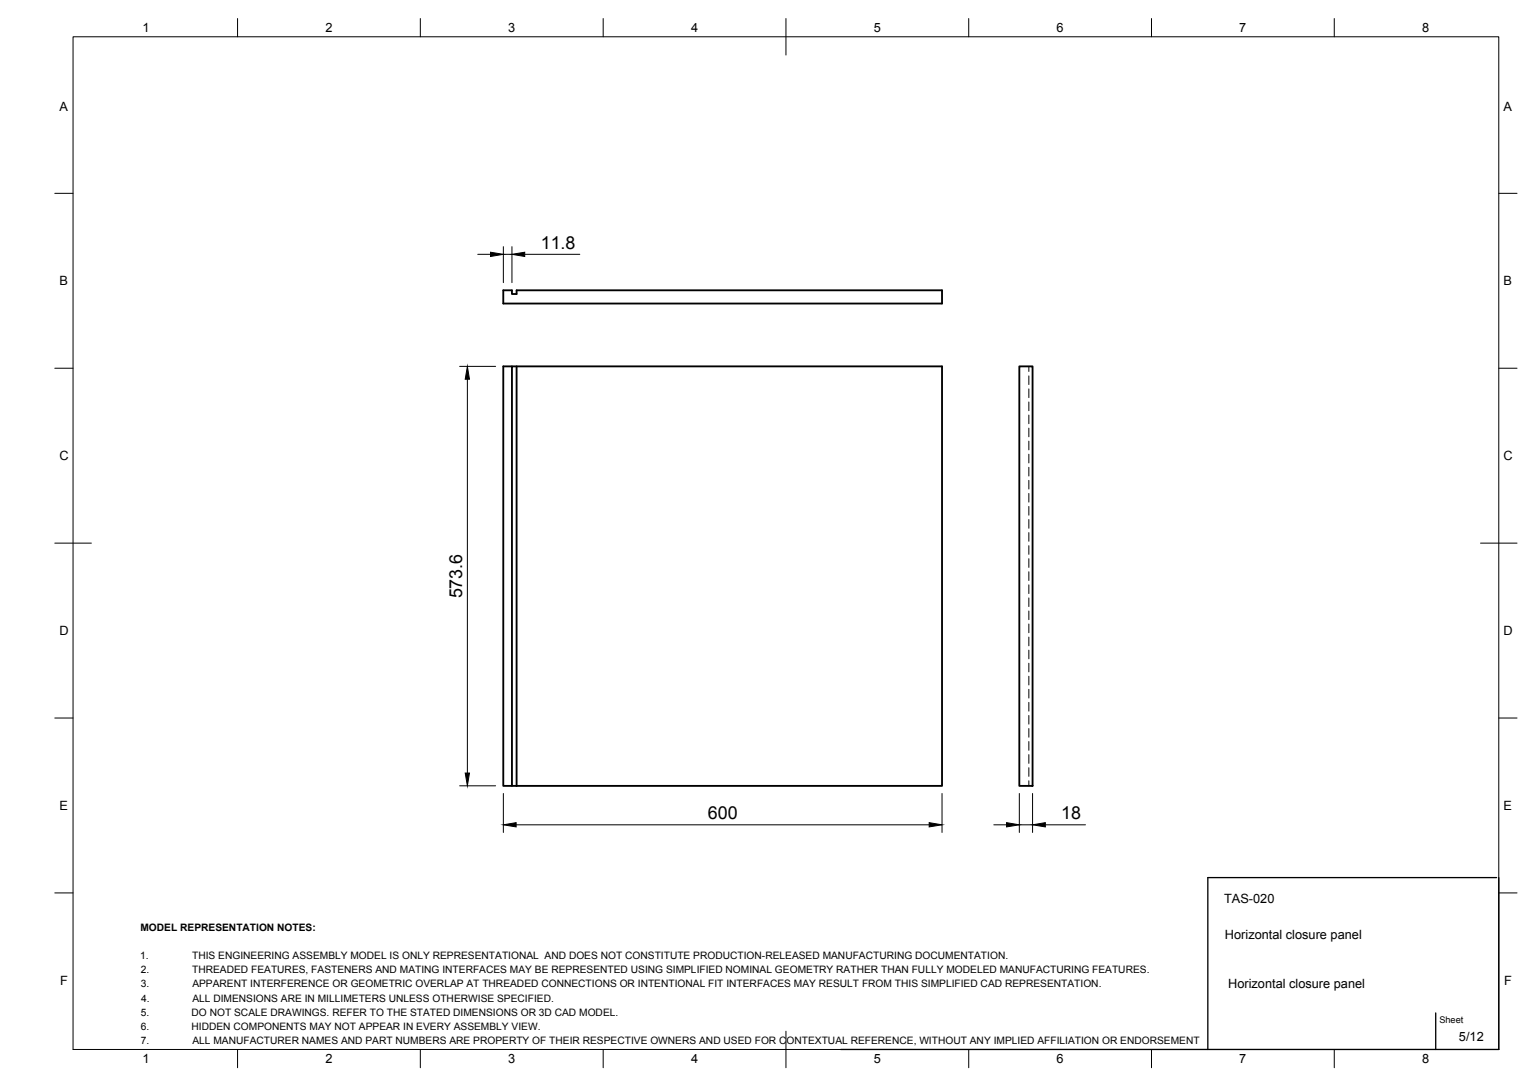
ISO-10303-21;
HEADER;
/* Generated by software containing ST-Developer
 * from STEP Tools, Inc. (www.steptools.com) 
 */

FILE_DESCRIPTION(
/* description */ (''),
/* implementation_level */ '2;1');

FILE_NAME(
/* name */ 'Horizontal closure panel.step',
/* time_stamp */ '2026-11-15T17:46:57-08:00',
/* author */ (''),
/* organization */ (''),
/* preprocessor_version */ 'ST-DEVELOPER v20.2',
/* originating_system */ 'Autodesk Translation Framework v15.17.0.0',
/* authorisation */ '');

FILE_SCHEMA (('AUTOMOTIVE_DESIGN { 1 0 10303 214 3 1 1 }'));
ENDSEC;

DATA;
#10=MECHANICAL_DESIGN_GEOMETRIC_PRESENTATION_REPRESENTATION('',(#377),#12963);
#353=SHAPE_REPRESENTATION_RELATIONSHIP('SRR','None',#13037,#365);
#365=ADVANCED_BREP_SHAPE_REPRESENTATION('',(#389),#12953);
#377=STYLED_ITEM('',(#13106),#389);
#389=MANIFOLD_SOLID_BREP('Body1',#4811);
#495=PLANE('',#5054);
#496=PLANE('',#5055);
#497=PLANE('',#5056);
#498=PLANE('',#5057);
#499=PLANE('',#5058);
#500=PLANE('',#5059);
#501=PLANE('',#5060);
#502=PLANE('',#5061);
#503=PLANE('',#5062);
#504=PLANE('',#5063);
#640=FACE_OUTER_BOUND('',#914,.T.);
#641=FACE_OUTER_BOUND('',#915,.T.);
#642=FACE_OUTER_BOUND('',#916,.T.);
#643=FACE_OUTER_BOUND('',#917,.T.);
#644=FACE_OUTER_BOUND('',#918,.T.);
#645=FACE_OUTER_BOUND('',#919,.T.);
#646=FACE_OUTER_BOUND('',#920,.T.);
#647=FACE_OUTER_BOUND('',#921,.T.);
#648=FACE_OUTER_BOUND('',#922,.T.);
#649=FACE_OUTER_BOUND('',#923,.T.);
#914=EDGE_LOOP('',(#3436,#3437,#3438,#3439));
#915=EDGE_LOOP('',(#3440,#3441,#3442,#3443));
#916=EDGE_LOOP('',(#3444,#3445,#3446,#3447));
#917=EDGE_LOOP('',(#3448,#3449,#3450,#3451,#3452,#3453,#3454,#3455));
#918=EDGE_LOOP('',(#3456,#3457,#3458,#3459));
#919=EDGE_LOOP('',(#3460,#3461,#3462,#3463));
#920=EDGE_LOOP('',(#3464,#3465,#3466,#3467));
#921=EDGE_LOOP('',(#3468,#3469,#3470,#3471,#3472,#3473,#3474,#3475));
#922=EDGE_LOOP('',(#3476,#3477,#3478,#3479));
#923=EDGE_LOOP('',(#3480,#3481,#3482,#3483));
#1260=LINE('',#6862,#1662);
#1261=LINE('',#6864,#1663);
#1262=LINE('',#6866,#1664);
#1263=LINE('',#6867,#1665);
#1264=LINE('',#6871,#1666);
#1265=LINE('',#6873,#1667);
#1266=LINE('',#6875,#1668);
#1267=LINE('',#6876,#1669);
#1268=LINE('',#6878,#1670);
#1269=LINE('',#6879,#1671);
#1270=LINE('',#6882,#1672);
#1271=LINE('',#6884,#1673);
#1272=LINE('',#6886,#1674);
#1273=LINE('',#6888,#1675);
#1274=LINE('',#6889,#1676);
#1275=LINE('',#6892,#1677);
#1276=LINE('',#6893,#1678);
#1277=LINE('',#6896,#1679);
#1278=LINE('',#6898,#1680);
#1279=LINE('',#6899,#1681);
#1280=LINE('',#6902,#1682);
#1281=LINE('',#6903,#1683);
#1282=LINE('',#6905,#1684);
#1283=LINE('',#6906,#1685);
#1662=VECTOR('',#5677,1.);
#1663=VECTOR('',#5678,1.);
#1664=VECTOR('',#5679,1.);
#1665=VECTOR('',#5680,1.);
#1666=VECTOR('',#5683,1.);
#1667=VECTOR('',#5684,1.);
#1668=VECTOR('',#5685,1.);
#1669=VECTOR('',#5686,1.);
#1670=VECTOR('',#5689,1.);
#1671=VECTOR('',#5690,1.);
#1672=VECTOR('',#5693,1.);
#1673=VECTOR('',#5694,1.);
#1674=VECTOR('',#5695,1.);
#1675=VECTOR('',#5696,1.);
#1676=VECTOR('',#5697,1.);
#1677=VECTOR('',#5700,1.);
#1678=VECTOR('',#5701,1.);
#1679=VECTOR('',#5704,1.);
#1680=VECTOR('',#5705,1.);
#1681=VECTOR('',#5706,1.);
#1682=VECTOR('',#5709,1.);
#1683=VECTOR('',#5710,1.);
#1684=VECTOR('',#5713,1.);
#1685=VECTOR('',#5714,1.);
#2120=VERTEX_POINT('',#6860);
#2121=VERTEX_POINT('',#6861);
#2122=VERTEX_POINT('',#6863);
#2123=VERTEX_POINT('',#6865);
#2124=VERTEX_POINT('',#6869);
#2125=VERTEX_POINT('',#6870);
#2126=VERTEX_POINT('',#6872);
#2127=VERTEX_POINT('',#6874);
#2128=VERTEX_POINT('',#6881);
#2129=VERTEX_POINT('',#6883);
#2130=VERTEX_POINT('',#6885);
#2131=VERTEX_POINT('',#6887);
#2132=VERTEX_POINT('',#6891);
#2133=VERTEX_POINT('',#6895);
#2134=VERTEX_POINT('',#6897);
#2135=VERTEX_POINT('',#6901);
#2614=EDGE_CURVE('',#2120,#2121,#1260,.T.);
#2615=EDGE_CURVE('',#2122,#2120,#1261,.T.);
#2616=EDGE_CURVE('',#2123,#2122,#1262,.T.);
#2617=EDGE_CURVE('',#2121,#2123,#1263,.T.);
#2618=EDGE_CURVE('',#2124,#2125,#1264,.T.);
#2619=EDGE_CURVE('',#2126,#2124,#1265,.T.);
#2620=EDGE_CURVE('',#2127,#2126,#1266,.T.);
#2621=EDGE_CURVE('',#2125,#2127,#1267,.T.);
#2622=EDGE_CURVE('',#2123,#2126,#1268,.T.);
#2623=EDGE_CURVE('',#2127,#2122,#1269,.T.);
#2624=EDGE_CURVE('',#2128,#2120,#1270,.T.);
#2625=EDGE_CURVE('',#2129,#2128,#1271,.T.);
#2626=EDGE_CURVE('',#2129,#2130,#1272,.T.);
#2627=EDGE_CURVE('',#2130,#2131,#1273,.T.);
#2628=EDGE_CURVE('',#2125,#2131,#1274,.T.);
#2629=EDGE_CURVE('',#2121,#2132,#1275,.T.);
#2630=EDGE_CURVE('',#2132,#2128,#1276,.T.);
#2631=EDGE_CURVE('',#2130,#2133,#1277,.T.);
#2632=EDGE_CURVE('',#2133,#2134,#1278,.T.);
#2633=EDGE_CURVE('',#2131,#2134,#1279,.T.);
#2634=EDGE_CURVE('',#2135,#2129,#1280,.T.);
#2635=EDGE_CURVE('',#2135,#2132,#1281,.T.);
#2636=EDGE_CURVE('',#2134,#2124,#1282,.T.);
#2637=EDGE_CURVE('',#2133,#2135,#1283,.T.);
#3436=ORIENTED_EDGE('',*,*,#2614,.F.);
#3437=ORIENTED_EDGE('',*,*,#2615,.F.);
#3438=ORIENTED_EDGE('',*,*,#2616,.F.);
#3439=ORIENTED_EDGE('',*,*,#2617,.F.);
#3440=ORIENTED_EDGE('',*,*,#2618,.F.);
#3441=ORIENTED_EDGE('',*,*,#2619,.F.);
#3442=ORIENTED_EDGE('',*,*,#2620,.F.);
#3443=ORIENTED_EDGE('',*,*,#2621,.F.);
#3444=ORIENTED_EDGE('',*,*,#2622,.F.);
#3445=ORIENTED_EDGE('',*,*,#2616,.T.);
#3446=ORIENTED_EDGE('',*,*,#2623,.F.);
#3447=ORIENTED_EDGE('',*,*,#2620,.T.);
#3448=ORIENTED_EDGE('',*,*,#2621,.T.);
#3449=ORIENTED_EDGE('',*,*,#2623,.T.);
#3450=ORIENTED_EDGE('',*,*,#2615,.T.);
#3451=ORIENTED_EDGE('',*,*,#2624,.F.);
#3452=ORIENTED_EDGE('',*,*,#2625,.F.);
#3453=ORIENTED_EDGE('',*,*,#2626,.T.);
#3454=ORIENTED_EDGE('',*,*,#2627,.T.);
#3455=ORIENTED_EDGE('',*,*,#2628,.F.);
#3456=ORIENTED_EDGE('',*,*,#2614,.T.);
#3457=ORIENTED_EDGE('',*,*,#2629,.T.);
#3458=ORIENTED_EDGE('',*,*,#2630,.T.);
#3459=ORIENTED_EDGE('',*,*,#2624,.T.);
#3460=ORIENTED_EDGE('',*,*,#2631,.T.);
#3461=ORIENTED_EDGE('',*,*,#2632,.T.);
#3462=ORIENTED_EDGE('',*,*,#2633,.F.);
#3463=ORIENTED_EDGE('',*,*,#2627,.F.);
#3464=ORIENTED_EDGE('',*,*,#2634,.T.);
#3465=ORIENTED_EDGE('',*,*,#2625,.T.);
#3466=ORIENTED_EDGE('',*,*,#2630,.F.);
#3467=ORIENTED_EDGE('',*,*,#2635,.F.);
#3468=ORIENTED_EDGE('',*,*,#2619,.T.);
#3469=ORIENTED_EDGE('',*,*,#2636,.F.);
#3470=ORIENTED_EDGE('',*,*,#2632,.F.);
#3471=ORIENTED_EDGE('',*,*,#2637,.T.);
#3472=ORIENTED_EDGE('',*,*,#2635,.T.);
#3473=ORIENTED_EDGE('',*,*,#2629,.F.);
#3474=ORIENTED_EDGE('',*,*,#2617,.T.);
#3475=ORIENTED_EDGE('',*,*,#2622,.T.);
#3476=ORIENTED_EDGE('',*,*,#2618,.T.);
#3477=ORIENTED_EDGE('',*,*,#2628,.T.);
#3478=ORIENTED_EDGE('',*,*,#2633,.T.);
#3479=ORIENTED_EDGE('',*,*,#2636,.T.);
#3480=ORIENTED_EDGE('',*,*,#2637,.F.);
#3481=ORIENTED_EDGE('',*,*,#2631,.F.);
#3482=ORIENTED_EDGE('',*,*,#2626,.F.);
#3483=ORIENTED_EDGE('',*,*,#2634,.F.);
#4621=ADVANCED_FACE('',(#640),#495,.F.);
#4622=ADVANCED_FACE('',(#641),#496,.F.);
#4623=ADVANCED_FACE('',(#642),#497,.T.);
#4624=ADVANCED_FACE('',(#643),#498,.T.);
#4625=ADVANCED_FACE('',(#644),#499,.T.);
#4626=ADVANCED_FACE('',(#645),#500,.T.);
#4627=ADVANCED_FACE('',(#646),#501,.T.);
#4628=ADVANCED_FACE('',(#647),#502,.T.);
#4629=ADVANCED_FACE('',(#648),#503,.T.);
#4630=ADVANCED_FACE('',(#649),#504,.F.);
#4811=CLOSED_SHELL('',(#4621,#4622,#4623,#4624,#4625,#4626,#4627,#4628,
#4629,#4630));
#5053=AXIS2_PLACEMENT_3D('',#6858,#5673,#5674);
#5054=AXIS2_PLACEMENT_3D('',#6859,#5675,#5676);
#5055=AXIS2_PLACEMENT_3D('',#6868,#5681,#5682);
#5056=AXIS2_PLACEMENT_3D('',#6877,#5687,#5688);
#5057=AXIS2_PLACEMENT_3D('',#6880,#5691,#5692);
#5058=AXIS2_PLACEMENT_3D('',#6890,#5698,#5699);
#5059=AXIS2_PLACEMENT_3D('',#6894,#5702,#5703);
#5060=AXIS2_PLACEMENT_3D('',#6900,#5707,#5708);
#5061=AXIS2_PLACEMENT_3D('',#6904,#5711,#5712);
#5062=AXIS2_PLACEMENT_3D('',#6907,#5715,#5716);
#5063=AXIS2_PLACEMENT_3D('',#6908,#5717,#5718);
#5673=DIRECTION('axis',(0.,0.,1.));
#5674=DIRECTION('refdir',(1.,0.,0.));
#5675=DIRECTION('center_axis',(0.,-1.,0.));
#5676=DIRECTION('ref_axis',(1.,0.,0.));
#5677=DIRECTION('',(-1.,0.,0.));
#5678=DIRECTION('',(0.,0.,1.));
#5679=DIRECTION('',(1.,0.,0.));
#5680=DIRECTION('',(0.,0.,-1.));
#5681=DIRECTION('center_axis',(0.,1.,0.));
#5682=DIRECTION('ref_axis',(-1.,0.,0.));
#5683=DIRECTION('',(1.,0.,0.));
#5684=DIRECTION('',(0.,0.,1.));
#5685=DIRECTION('',(-1.,0.,0.));
#5686=DIRECTION('',(0.,0.,-1.));
#5687=DIRECTION('center_axis',(0.,0.,1.));
#5688=DIRECTION('ref_axis',(1.,0.,0.));
#5689=DIRECTION('',(0.,1.,0.));
#5690=DIRECTION('',(0.,-1.,0.));
#5691=DIRECTION('center_axis',(1.,0.,0.));
#5692=DIRECTION('ref_axis',(0.,1.,0.));
#5693=DIRECTION('',(0.,1.,0.));
#5694=DIRECTION('',(0.,0.,1.));
#5695=DIRECTION('',(0.,1.,0.));
#5696=DIRECTION('',(0.,0.,1.));
#5697=DIRECTION('',(0.,1.,0.));
#5698=DIRECTION('center_axis',(0.,0.,1.));
#5699=DIRECTION('ref_axis',(1.,0.,0.));
#5700=DIRECTION('',(0.,-1.,0.));
#5701=DIRECTION('',(1.,0.,0.));
#5702=DIRECTION('center_axis',(0.,1.,0.));
#5703=DIRECTION('ref_axis',(-1.,0.,0.));
#5704=DIRECTION('',(-1.,0.,0.));
#5705=DIRECTION('',(0.,0.,1.));
#5706=DIRECTION('',(-1.,0.,0.));
#5707=DIRECTION('center_axis',(0.,-1.,0.));
#5708=DIRECTION('ref_axis',(1.,0.,0.));
#5709=DIRECTION('',(1.,0.,0.));
#5710=DIRECTION('',(0.,0.,1.));
#5711=DIRECTION('center_axis',(-1.,0.,0.));
#5712=DIRECTION('ref_axis',(0.,-1.,0.));
#5713=DIRECTION('',(0.,-1.,0.));
#5714=DIRECTION('',(0.,-1.,0.));
#5715=DIRECTION('center_axis',(0.,0.,1.));
#5716=DIRECTION('ref_axis',(1.,0.,0.));
#5717=DIRECTION('center_axis',(0.,0.,1.));
#5718=DIRECTION('ref_axis',(1.,0.,0.));
#6858=CARTESIAN_POINT('',(0.,0.,0.));
#6859=CARTESIAN_POINT('Origin',(0.,58.18,1.3));
#6860=CARTESIAN_POINT('',(57.36,58.18,1.8));
#6861=CARTESIAN_POINT('',(0.,58.18,1.8));
#6862=CARTESIAN_POINT('',(14.34,58.18,1.8));
#6863=CARTESIAN_POINT('',(57.36,58.18,1.3));
#6864=CARTESIAN_POINT('',(57.36,58.18,0.65));
#6865=CARTESIAN_POINT('',(0.,58.18,1.3));
#6866=CARTESIAN_POINT('',(0.,58.18,1.3));
#6867=CARTESIAN_POINT('',(0.,58.18,0.65));
#6868=CARTESIAN_POINT('Origin',(57.36,58.82,1.3));
#6869=CARTESIAN_POINT('',(0.,58.82,1.8));
#6870=CARTESIAN_POINT('',(57.36,58.82,1.8));
#6871=CARTESIAN_POINT('',(43.02,58.82,1.8));
#6872=CARTESIAN_POINT('',(0.,58.82,1.3));
#6873=CARTESIAN_POINT('',(0.,58.82,0.65));
#6874=CARTESIAN_POINT('',(57.36,58.82,1.3));
#6875=CARTESIAN_POINT('',(57.36,58.82,1.3));
#6876=CARTESIAN_POINT('',(57.36,58.82,0.65));
#6877=CARTESIAN_POINT('Origin',(28.68,58.5,1.3));
#6878=CARTESIAN_POINT('',(0.,59.25,1.3));
#6879=CARTESIAN_POINT('',(57.36,29.25,1.3));
#6880=CARTESIAN_POINT('Origin',(57.36,0.,0.));
#6881=CARTESIAN_POINT('',(57.36,0.,1.8));
#6882=CARTESIAN_POINT('',(57.36,0.,1.8));
#6883=CARTESIAN_POINT('',(57.36,0.,0.));
#6884=CARTESIAN_POINT('',(57.36,0.,0.));
#6885=CARTESIAN_POINT('',(57.36,60.,0.));
#6886=CARTESIAN_POINT('',(57.36,0.,0.));
#6887=CARTESIAN_POINT('',(57.36,60.,1.8));
#6888=CARTESIAN_POINT('',(57.36,60.,0.));
#6889=CARTESIAN_POINT('',(57.36,0.,1.8));
#6890=CARTESIAN_POINT('Origin',(28.68,30.,1.8));
#6891=CARTESIAN_POINT('',(0.,0.,1.8));
#6892=CARTESIAN_POINT('',(0.,60.,1.8));
#6893=CARTESIAN_POINT('',(0.,0.,1.8));
#6894=CARTESIAN_POINT('Origin',(57.36,60.,0.));
#6895=CARTESIAN_POINT('',(0.,60.,0.));
#6896=CARTESIAN_POINT('',(57.36,60.,0.));
#6897=CARTESIAN_POINT('',(0.,60.,1.8));
#6898=CARTESIAN_POINT('',(0.,60.,0.));
#6899=CARTESIAN_POINT('',(57.36,60.,1.8));
#6900=CARTESIAN_POINT('Origin',(0.,0.,0.));
#6901=CARTESIAN_POINT('',(0.,0.,0.));
#6902=CARTESIAN_POINT('',(0.,0.,0.));
#6903=CARTESIAN_POINT('',(0.,0.,0.));
#6904=CARTESIAN_POINT('Origin',(0.,60.,0.));
#6905=CARTESIAN_POINT('',(0.,60.,1.8));
#6906=CARTESIAN_POINT('',(0.,60.,0.));
#6907=CARTESIAN_POINT('Origin',(28.68,30.,1.8));
#6908=CARTESIAN_POINT('Origin',(28.68,30.,0.));
#12939=UNCERTAINTY_MEASURE_WITH_UNIT(LENGTH_MEASURE(0.001),#12964,
'DISTANCE_ACCURACY_VALUE',
'Maximum model space distance between geometric entities at asserted c
onnectivities');
#12949=UNCERTAINTY_MEASURE_WITH_UNIT(LENGTH_MEASURE(0.001),#12964,
'DISTANCE_ACCURACY_VALUE',
'Maximum model space distance between geometric entities at asserted c
onnectivities');
#12953=(
GEOMETRIC_REPRESENTATION_CONTEXT(3)
GLOBAL_UNCERTAINTY_ASSIGNED_CONTEXT((#12939))
GLOBAL_UNIT_ASSIGNED_CONTEXT((#12964,#12966,#12967))
REPRESENTATION_CONTEXT('','3D')
);
#12963=(
GEOMETRIC_REPRESENTATION_CONTEXT(3)
GLOBAL_UNCERTAINTY_ASSIGNED_CONTEXT((#12949))
GLOBAL_UNIT_ASSIGNED_CONTEXT((#12964,#12966,#12967))
REPRESENTATION_CONTEXT('','3D')
);
#12964=(
LENGTH_UNIT()
NAMED_UNIT(*)
SI_UNIT(.CENTI.,.METRE.)
);
#12966=(
NAMED_UNIT(*)
PLANE_ANGLE_UNIT()
SI_UNIT($,.RADIAN.)
);
#12967=(
NAMED_UNIT(*)
SI_UNIT($,.STERADIAN.)
SOLID_ANGLE_UNIT()
);
#12971=SHAPE_DEFINITION_REPRESENTATION(#12984,#13037);
#12984=PRODUCT_DEFINITION_SHAPE('',$,#13051);
#13037=SHAPE_REPRESENTATION('',(#5053),#12953);
#13047=PRODUCT_DEFINITION_CONTEXT('part definition',#13088,'design');
#13051=PRODUCT_DEFINITION('Horizontal closure panel',
'Horizontal closure panel',#13064,#13047);
#13064=PRODUCT_DEFINITION_FORMATION('',$,#13093);
#13088=APPLICATION_CONTEXT(
'Core Data for Automotive Mechanical Design Process');
#13089=PRODUCT_CONTEXT('part definition',#13088,'mechanical');
#13093=PRODUCT('Horizontal closure panel','Horizontal closure panel',$,
(#13089));
#13106=PRESENTATION_STYLE_ASSIGNMENT((#13119));
#13119=SURFACE_STYLE_USAGE(.BOTH.,#13132);
#13132=SURFACE_SIDE_STYLE('',(#13145));
#13145=SURFACE_STYLE_FILL_AREA(#13158);
#13158=FILL_AREA_STYLE('Horizontal closure panel finish',(#13171));
#13171=FILL_AREA_STYLE_COLOUR('Horizontal closure panel finish',#13184);
#13184=COLOUR_RGB('Horizontal closure panel finish',0.662745098039216,0.823529411764706,
0.917647058823529);
ENDSEC;
END-ISO-10303-21;
